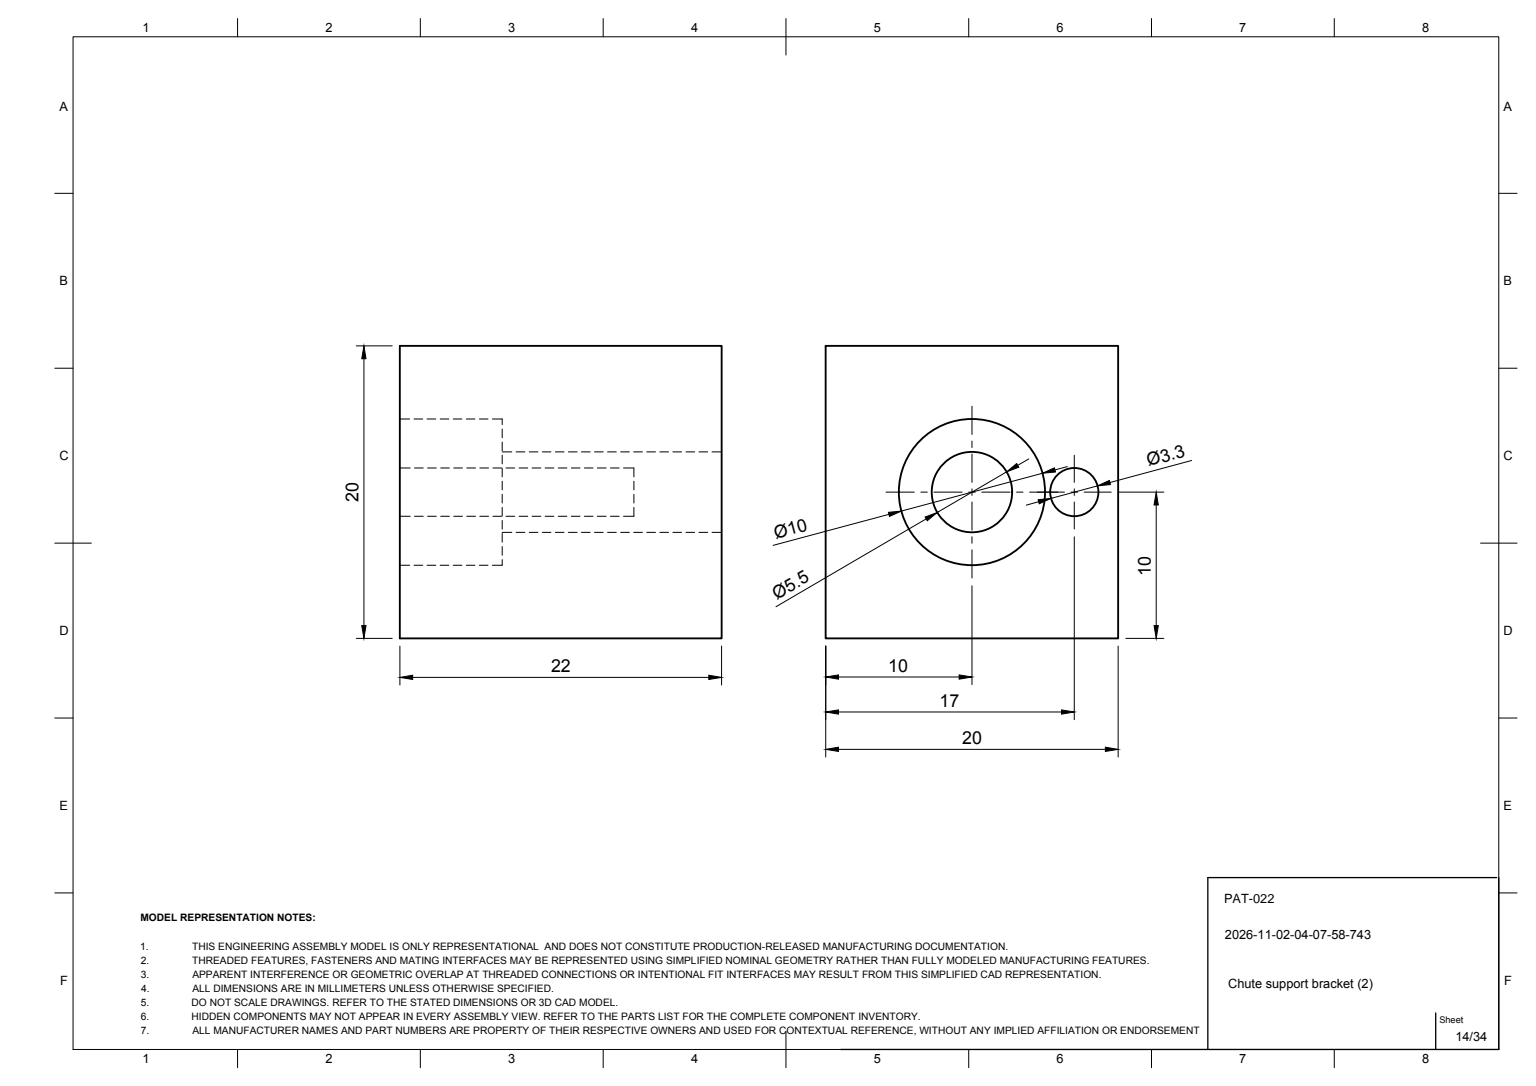
ISO-10303-21;
HEADER;
/* Generated by software containing ST-Developer
 * from STEP Tools, Inc. (www.steptools.com) 
 */

FILE_DESCRIPTION(
/* description */ ('Chute with adjustable gate'),
/* implementation_level */ '2;1');

FILE_NAME(
/* name */ 'Chute support bracket (2).step',
/* time_stamp */ '2026-10-27T10:52:28-07:00',
/* author */ (''),
/* organization */ (''),
/* preprocessor_version */ 'ST-DEVELOPER v20.2',
/* originating_system */ 'Autodesk Translation Framework v15.17.0.0',
/* authorisation */ '');

FILE_SCHEMA (('AUTOMOTIVE_DESIGN { 1 0 10303 214 3 1 1 }'));
ENDSEC;

DATA;
#10=MECHANICAL_DESIGN_GEOMETRIC_PRESENTATION_REPRESENTATION('',(#423),#13094);
#359=SHAPE_REPRESENTATION_RELATIONSHIP('SRR','None',#13260,#391);
#391=ADVANCED_BREP_SHAPE_REPRESENTATION('',(#455),#13069);
#423=STYLED_ITEM('',(#13474),#455);
#455=MANIFOLD_SOLID_BREP('Body1',#7606);
#508=FACE_BOUND('',#1447,.T.);
#509=FACE_BOUND('',#1450,.T.);
#510=FACE_BOUND('',#1451,.T.);
#511=FACE_BOUND('',#1454,.T.);
#652=PLANE('',#8117);
#653=PLANE('',#8121);
#654=PLANE('',#8125);
#655=PLANE('',#8126);
#656=PLANE('',#8127);
#657=PLANE('',#8128);
#658=PLANE('',#8129);
#659=PLANE('',#8130);
#994=FACE_OUTER_BOUND('',#1443,.T.);
#995=FACE_OUTER_BOUND('',#1444,.T.);
#996=FACE_OUTER_BOUND('',#1445,.T.);
#997=FACE_OUTER_BOUND('',#1446,.T.);
#998=FACE_OUTER_BOUND('',#1448,.T.);
#999=FACE_OUTER_BOUND('',#1449,.T.);
#1000=FACE_OUTER_BOUND('',#1452,.T.);
#1001=FACE_OUTER_BOUND('',#1453,.T.);
#1002=FACE_OUTER_BOUND('',#1455,.T.);
#1003=FACE_OUTER_BOUND('',#1456,.T.);
#1004=FACE_OUTER_BOUND('',#1457,.T.);
#1443=EDGE_LOOP('',(#5534,#5535,#5536,#5537));
#1444=EDGE_LOOP('',(#5538));
#1445=EDGE_LOOP('',(#5539,#5540,#5541,#5542));
#1446=EDGE_LOOP('',(#5543));
#1447=EDGE_LOOP('',(#5544));
#1448=EDGE_LOOP('',(#5545,#5546,#5547,#5548));
#1449=EDGE_LOOP('',(#5549,#5550,#5551,#5552));
#1450=EDGE_LOOP('',(#5553));
#1451=EDGE_LOOP('',(#5554));
#1452=EDGE_LOOP('',(#5555,#5556,#5557,#5558));
#1453=EDGE_LOOP('',(#5559,#5560,#5561,#5562));
#1454=EDGE_LOOP('',(#5563));
#1455=EDGE_LOOP('',(#5564,#5565,#5566,#5567));
#1456=EDGE_LOOP('',(#5568,#5569,#5570,#5571));
#1457=EDGE_LOOP('',(#5572,#5573,#5574,#5575));
#1998=LINE('',#11285,#2775);
#1999=LINE('',#11292,#2776);
#2000=LINE('',#11300,#2777);
#2001=LINE('',#11304,#2778);
#2002=LINE('',#11306,#2779);
#2003=LINE('',#11308,#2780);
#2004=LINE('',#11309,#2781);
#2005=LINE('',#11312,#2782);
#2006=LINE('',#11314,#2783);
#2007=LINE('',#11315,#2784);
#2008=LINE('',#11318,#2785);
#2009=LINE('',#11320,#2786);
#2010=LINE('',#11321,#2787);
#2011=LINE('',#11323,#2788);
#2012=LINE('',#11324,#2789);
#2775=VECTOR('',#9096,0.164999999999999);
#2776=VECTOR('',#9105,0.5);
#2777=VECTOR('',#9116,0.274999999999999);
#2778=VECTOR('',#9119,1.);
#2779=VECTOR('',#9120,1.);
#2780=VECTOR('',#9121,1.);
#2781=VECTOR('',#9122,1.);
#2782=VECTOR('',#9125,1.);
#2783=VECTOR('',#9126,1.);
#2784=VECTOR('',#9127,1.);
#2785=VECTOR('',#9130,1.);
#2786=VECTOR('',#9131,1.);
#2787=VECTOR('',#9132,1.);
#2788=VECTOR('',#9135,1.);
#2789=VECTOR('',#9136,1.);
#3450=CIRCLE('',#8115,0.164999999999999);
#3451=CIRCLE('',#8116,0.164999999999999);
#3452=CIRCLE('',#8119,0.5);
#3453=CIRCLE('',#8120,0.5);
#3454=CIRCLE('',#8122,0.274999999999999);
#3455=CIRCLE('',#8124,0.274999999999999);
#3709=VERTEX_POINT('',#11282);
#3710=VERTEX_POINT('',#11284);
#3711=VERTEX_POINT('',#11289);
#3712=VERTEX_POINT('',#11291);
#3713=VERTEX_POINT('',#11295);
#3714=VERTEX_POINT('',#11298);
#3715=VERTEX_POINT('',#11302);
#3716=VERTEX_POINT('',#11303);
#3717=VERTEX_POINT('',#11305);
#3718=VERTEX_POINT('',#11307);
#3719=VERTEX_POINT('',#11311);
#3720=VERTEX_POINT('',#11313);
#3721=VERTEX_POINT('',#11317);
#3722=VERTEX_POINT('',#11319);
#4400=EDGE_CURVE('',#3709,#3709,#3450,.T.);
#4401=EDGE_CURVE('',#3709,#3710,#1998,.T.);
#4402=EDGE_CURVE('',#3710,#3710,#3451,.T.);
#4403=EDGE_CURVE('',#3711,#3711,#3452,.T.);
#4404=EDGE_CURVE('',#3711,#3712,#1999,.T.);
#4405=EDGE_CURVE('',#3712,#3712,#3453,.T.);
#4406=EDGE_CURVE('',#3713,#3713,#3454,.T.);
#4407=EDGE_CURVE('',#3714,#3714,#3455,.T.);
#4408=EDGE_CURVE('',#3714,#3713,#2000,.T.);
#4409=EDGE_CURVE('',#3715,#3716,#2001,.T.);
#4410=EDGE_CURVE('',#3716,#3717,#2002,.T.);
#4411=EDGE_CURVE('',#3718,#3717,#2003,.T.);
#4412=EDGE_CURVE('',#3715,#3718,#2004,.T.);
#4413=EDGE_CURVE('',#3719,#3715,#2005,.T.);
#4414=EDGE_CURVE('',#3720,#3718,#2006,.T.);
#4415=EDGE_CURVE('',#3719,#3720,#2007,.T.);
#4416=EDGE_CURVE('',#3721,#3719,#2008,.T.);
#4417=EDGE_CURVE('',#3722,#3720,#2009,.T.);
#4418=EDGE_CURVE('',#3721,#3722,#2010,.T.);
#4419=EDGE_CURVE('',#3716,#3721,#2011,.T.);
#4420=EDGE_CURVE('',#3717,#3722,#2012,.T.);
#5534=ORIENTED_EDGE('',*,*,#4400,.F.);
#5535=ORIENTED_EDGE('',*,*,#4401,.T.);
#5536=ORIENTED_EDGE('',*,*,#4402,.F.);
#5537=ORIENTED_EDGE('',*,*,#4401,.F.);
#5538=ORIENTED_EDGE('',*,*,#4400,.T.);
#5539=ORIENTED_EDGE('',*,*,#4403,.F.);
#5540=ORIENTED_EDGE('',*,*,#4404,.T.);
#5541=ORIENTED_EDGE('',*,*,#4405,.F.);
#5542=ORIENTED_EDGE('',*,*,#4404,.F.);
#5543=ORIENTED_EDGE('',*,*,#4403,.T.);
#5544=ORIENTED_EDGE('',*,*,#4406,.F.);
#5545=ORIENTED_EDGE('',*,*,#4407,.F.);
#5546=ORIENTED_EDGE('',*,*,#4408,.T.);
#5547=ORIENTED_EDGE('',*,*,#4406,.T.);
#5548=ORIENTED_EDGE('',*,*,#4408,.F.);
#5549=ORIENTED_EDGE('',*,*,#4409,.T.);
#5550=ORIENTED_EDGE('',*,*,#4410,.T.);
#5551=ORIENTED_EDGE('',*,*,#4411,.F.);
#5552=ORIENTED_EDGE('',*,*,#4412,.F.);
#5553=ORIENTED_EDGE('',*,*,#4402,.T.);
#5554=ORIENTED_EDGE('',*,*,#4405,.T.);
#5555=ORIENTED_EDGE('',*,*,#4413,.T.);
#5556=ORIENTED_EDGE('',*,*,#4412,.T.);
#5557=ORIENTED_EDGE('',*,*,#4414,.F.);
#5558=ORIENTED_EDGE('',*,*,#4415,.F.);
#5559=ORIENTED_EDGE('',*,*,#4416,.T.);
#5560=ORIENTED_EDGE('',*,*,#4415,.T.);
#5561=ORIENTED_EDGE('',*,*,#4417,.F.);
#5562=ORIENTED_EDGE('',*,*,#4418,.F.);
#5563=ORIENTED_EDGE('',*,*,#4407,.T.);
#5564=ORIENTED_EDGE('',*,*,#4419,.T.);
#5565=ORIENTED_EDGE('',*,*,#4418,.T.);
#5566=ORIENTED_EDGE('',*,*,#4420,.F.);
#5567=ORIENTED_EDGE('',*,*,#4410,.F.);
#5568=ORIENTED_EDGE('',*,*,#4420,.T.);
#5569=ORIENTED_EDGE('',*,*,#4417,.T.);
#5570=ORIENTED_EDGE('',*,*,#4414,.T.);
#5571=ORIENTED_EDGE('',*,*,#4411,.T.);
#5572=ORIENTED_EDGE('',*,*,#4419,.F.);
#5573=ORIENTED_EDGE('',*,*,#4409,.F.);
#5574=ORIENTED_EDGE('',*,*,#4413,.F.);
#5575=ORIENTED_EDGE('',*,*,#4416,.F.);
#7124=CYLINDRICAL_SURFACE('',#8114,0.164999999999999);
#7125=CYLINDRICAL_SURFACE('',#8118,0.5);
#7126=CYLINDRICAL_SURFACE('',#8123,0.274999999999999);
#7262=ADVANCED_FACE('',(#994),#7124,.F.);
#7263=ADVANCED_FACE('',(#995),#652,.T.);
#7264=ADVANCED_FACE('',(#996),#7125,.F.);
#7265=ADVANCED_FACE('',(#997,#508),#653,.T.);
#7266=ADVANCED_FACE('',(#998),#7126,.F.);
#7267=ADVANCED_FACE('',(#999,#509,#510),#654,.T.);
#7268=ADVANCED_FACE('',(#1000),#655,.T.);
#7269=ADVANCED_FACE('',(#1001,#511),#656,.T.);
#7270=ADVANCED_FACE('',(#1002),#657,.T.);
#7271=ADVANCED_FACE('',(#1003),#658,.T.);
#7272=ADVANCED_FACE('',(#1004),#659,.F.);
#7606=CLOSED_SHELL('',(#7262,#7263,#7264,#7265,#7266,#7267,#7268,#7269,
#7270,#7271,#7272));
#8113=AXIS2_PLACEMENT_3D('',#11280,#9090,#9091);
#8114=AXIS2_PLACEMENT_3D('',#11281,#9092,#9093);
#8115=AXIS2_PLACEMENT_3D('',#11283,#9094,#9095);
#8116=AXIS2_PLACEMENT_3D('',#11286,#9097,#9098);
#8117=AXIS2_PLACEMENT_3D('',#11287,#9099,#9100);
#8118=AXIS2_PLACEMENT_3D('',#11288,#9101,#9102);
#8119=AXIS2_PLACEMENT_3D('',#11290,#9103,#9104);
#8120=AXIS2_PLACEMENT_3D('',#11293,#9106,#9107);
#8121=AXIS2_PLACEMENT_3D('',#11294,#9108,#9109);
#8122=AXIS2_PLACEMENT_3D('',#11296,#9110,#9111);
#8123=AXIS2_PLACEMENT_3D('',#11297,#9112,#9113);
#8124=AXIS2_PLACEMENT_3D('',#11299,#9114,#9115);
#8125=AXIS2_PLACEMENT_3D('',#11301,#9117,#9118);
#8126=AXIS2_PLACEMENT_3D('',#11310,#9123,#9124);
#8127=AXIS2_PLACEMENT_3D('',#11316,#9128,#9129);
#8128=AXIS2_PLACEMENT_3D('',#11322,#9133,#9134);
#8129=AXIS2_PLACEMENT_3D('',#11325,#9137,#9138);
#8130=AXIS2_PLACEMENT_3D('',#11326,#9139,#9140);
#9090=DIRECTION('axis',(0.,0.,1.));
#9091=DIRECTION('refdir',(1.,0.,0.));
#9092=DIRECTION('center_axis',(0.,1.,0.));
#9093=DIRECTION('ref_axis',(1.,0.,0.));
#9094=DIRECTION('center_axis',(0.,1.,0.));
#9095=DIRECTION('ref_axis',(1.,0.,0.));
#9096=DIRECTION('',(0.,1.,0.));
#9097=DIRECTION('center_axis',(0.,-1.,0.));
#9098=DIRECTION('ref_axis',(1.,0.,0.));
#9099=DIRECTION('center_axis',(0.,1.,0.));
#9100=DIRECTION('ref_axis',(1.,0.,0.));
#9101=DIRECTION('center_axis',(0.,1.,0.));
#9102=DIRECTION('ref_axis',(1.,0.,0.));
#9103=DIRECTION('center_axis',(0.,1.,0.));
#9104=DIRECTION('ref_axis',(1.,0.,0.));
#9105=DIRECTION('',(0.,1.,0.));
#9106=DIRECTION('center_axis',(0.,-1.,0.));
#9107=DIRECTION('ref_axis',(1.,0.,0.));
#9108=DIRECTION('center_axis',(0.,1.,0.));
#9109=DIRECTION('ref_axis',(1.,0.,0.));
#9110=DIRECTION('center_axis',(0.,1.,0.));
#9111=DIRECTION('ref_axis',(1.,0.,0.));
#9112=DIRECTION('center_axis',(0.,1.,0.));
#9113=DIRECTION('ref_axis',(1.,0.,0.));
#9114=DIRECTION('center_axis',(0.,1.,0.));
#9115=DIRECTION('ref_axis',(1.,0.,0.));
#9116=DIRECTION('',(0.,1.,0.));
#9117=DIRECTION('center_axis',(0.,1.,0.));
#9118=DIRECTION('ref_axis',(-1.,0.,0.));
#9119=DIRECTION('',(-1.,0.,0.));
#9120=DIRECTION('',(0.,0.,1.));
#9121=DIRECTION('',(-1.,0.,0.));
#9122=DIRECTION('',(0.,0.,1.));
#9123=DIRECTION('center_axis',(1.,0.,0.));
#9124=DIRECTION('ref_axis',(0.,1.,0.));
#9125=DIRECTION('',(0.,1.,0.));
#9126=DIRECTION('',(0.,1.,0.));
#9127=DIRECTION('',(0.,0.,1.));
#9128=DIRECTION('center_axis',(0.,-1.,0.));
#9129=DIRECTION('ref_axis',(1.,0.,0.));
#9130=DIRECTION('',(1.,0.,0.));
#9131=DIRECTION('',(1.,0.,0.));
#9132=DIRECTION('',(0.,0.,1.));
#9133=DIRECTION('center_axis',(-1.,0.,0.));
#9134=DIRECTION('ref_axis',(0.,-1.,0.));
#9135=DIRECTION('',(0.,-1.,0.));
#9136=DIRECTION('',(0.,-1.,0.));
#9137=DIRECTION('center_axis',(0.,0.,1.));
#9138=DIRECTION('ref_axis',(1.,0.,0.));
#9139=DIRECTION('center_axis',(0.,0.,1.));
#9140=DIRECTION('ref_axis',(1.,0.,0.));
#11280=CARTESIAN_POINT('',(0.,0.,0.));
#11281=CARTESIAN_POINT('Origin',(22.3,-9.4,12.));
#11282=CARTESIAN_POINT('',(22.135,-9.4,12.));
#11283=CARTESIAN_POINT('Origin',(22.3,-9.4,12.));
#11284=CARTESIAN_POINT('',(22.135,-7.8,12.));
#11285=CARTESIAN_POINT('',(22.135,-9.4,12.));
#11286=CARTESIAN_POINT('Origin',(22.3,-7.8,12.));
#11287=CARTESIAN_POINT('Origin',(22.3,-9.4,12.));
#11288=CARTESIAN_POINT('Origin',(23.,-8.5,12.));
#11289=CARTESIAN_POINT('',(22.5,-8.5,12.));
#11290=CARTESIAN_POINT('Origin',(23.,-8.5,12.));
#11291=CARTESIAN_POINT('',(22.5,-7.8,12.));
#11292=CARTESIAN_POINT('',(22.5,-8.5,12.));
#11293=CARTESIAN_POINT('Origin',(23.,-7.8,12.));
#11294=CARTESIAN_POINT('Origin',(23.,-8.5,12.));
#11295=CARTESIAN_POINT('',(22.725,-8.5,12.));
#11296=CARTESIAN_POINT('Origin',(23.,-8.5,12.));
#11297=CARTESIAN_POINT('Origin',(23.,-10.1,12.));
#11298=CARTESIAN_POINT('',(22.725,-10.,12.));
#11299=CARTESIAN_POINT('Origin',(23.,-10.,12.));
#11300=CARTESIAN_POINT('',(22.725,-10.1,12.));
#11301=CARTESIAN_POINT('Origin',(24.,-7.8,11.));
#11302=CARTESIAN_POINT('',(24.,-7.8,11.));
#11303=CARTESIAN_POINT('',(22.,-7.8,11.));
#11304=CARTESIAN_POINT('',(24.,-7.8,11.));
#11305=CARTESIAN_POINT('',(22.,-7.8,13.));
#11306=CARTESIAN_POINT('',(22.,-7.8,11.));
#11307=CARTESIAN_POINT('',(24.,-7.8,13.));
#11308=CARTESIAN_POINT('',(24.,-7.8,13.));
#11309=CARTESIAN_POINT('',(24.,-7.8,11.));
#11310=CARTESIAN_POINT('Origin',(24.,-10.,11.));
#11311=CARTESIAN_POINT('',(24.,-10.,11.));
#11312=CARTESIAN_POINT('',(24.,-10.,11.));
#11313=CARTESIAN_POINT('',(24.,-10.,13.));
#11314=CARTESIAN_POINT('',(24.,-10.,13.));
#11315=CARTESIAN_POINT('',(24.,-10.,11.));
#11316=CARTESIAN_POINT('Origin',(22.,-10.,11.));
#11317=CARTESIAN_POINT('',(22.,-10.,11.));
#11318=CARTESIAN_POINT('',(22.,-10.,11.));
#11319=CARTESIAN_POINT('',(22.,-10.,13.));
#11320=CARTESIAN_POINT('',(22.,-10.,13.));
#11321=CARTESIAN_POINT('',(22.,-10.,11.));
#11322=CARTESIAN_POINT('Origin',(22.,-7.8,11.));
#11323=CARTESIAN_POINT('',(22.,-7.8,11.));
#11324=CARTESIAN_POINT('',(22.,-7.8,13.));
#11325=CARTESIAN_POINT('Origin',(23.,-8.9,13.));
#11326=CARTESIAN_POINT('Origin',(23.,-8.9,11.));
#13032=UNCERTAINTY_MEASURE_WITH_UNIT(LENGTH_MEASURE(0.001),#13095,
'DISTANCE_ACCURACY_VALUE',
'Maximum model space distance between geometric entities at asserted c
onnectivities');
#13057=UNCERTAINTY_MEASURE_WITH_UNIT(LENGTH_MEASURE(0.001),#13095,
'DISTANCE_ACCURACY_VALUE',
'Maximum model space distance between geometric entities at asserted c
onnectivities');
#13069=(
GEOMETRIC_REPRESENTATION_CONTEXT(3)
GLOBAL_UNCERTAINTY_ASSIGNED_CONTEXT((#13032))
GLOBAL_UNIT_ASSIGNED_CONTEXT((#13095,#13097,#13098))
REPRESENTATION_CONTEXT('','3D')
);
#13094=(
GEOMETRIC_REPRESENTATION_CONTEXT(3)
GLOBAL_UNCERTAINTY_ASSIGNED_CONTEXT((#13057))
GLOBAL_UNIT_ASSIGNED_CONTEXT((#13095,#13097,#13098))
REPRESENTATION_CONTEXT('','3D')
);
#13095=(
LENGTH_UNIT()
NAMED_UNIT(*)
SI_UNIT(.CENTI.,.METRE.)
);
#13097=(
NAMED_UNIT(*)
PLANE_ANGLE_UNIT()
SI_UNIT($,.RADIAN.)
);
#13098=(
NAMED_UNIT(*)
SI_UNIT($,.STERADIAN.)
SOLID_ANGLE_UNIT()
);
#13110=SHAPE_DEFINITION_REPRESENTATION(#13146,#13260);
#13146=PRODUCT_DEFINITION_SHAPE('',$,#13297);
#13260=SHAPE_REPRESENTATION('',(#8113),#13069);
#13285=PRODUCT_DEFINITION_CONTEXT('part definition',#13395,'design');
#13297=PRODUCT_DEFINITION('Chute support bracket (2)',
'Chute support bracket (2)',#13333,#13285);
#13333=PRODUCT_DEFINITION_FORMATION('',$,#13408);
#13395=APPLICATION_CONTEXT(
'Core Data for Automotive Mechanical Design Process');
#13396=PRODUCT_CONTEXT('part definition',#13395,'mechanical');
#13408=PRODUCT('Chute support bracket (2)','Chute support bracket (2)',
'Chute support bracket (2)',(#13396));
#13468=COLOUR_RGB('Dark Blue',0.08,0.2,0.34);
#13469=FILL_AREA_STYLE_COLOUR('',#13468);
#13470=FILL_AREA_STYLE('',(#13469));
#13471=SURFACE_STYLE_FILL_AREA(#13470);
#13472=SURFACE_SIDE_STYLE('',(#13471));
#13473=SURFACE_STYLE_USAGE(.BOTH.,#13472);
#13474=PRESENTATION_STYLE_ASSIGNMENT((#13473));
ENDSEC;
END-ISO-10303-21;
